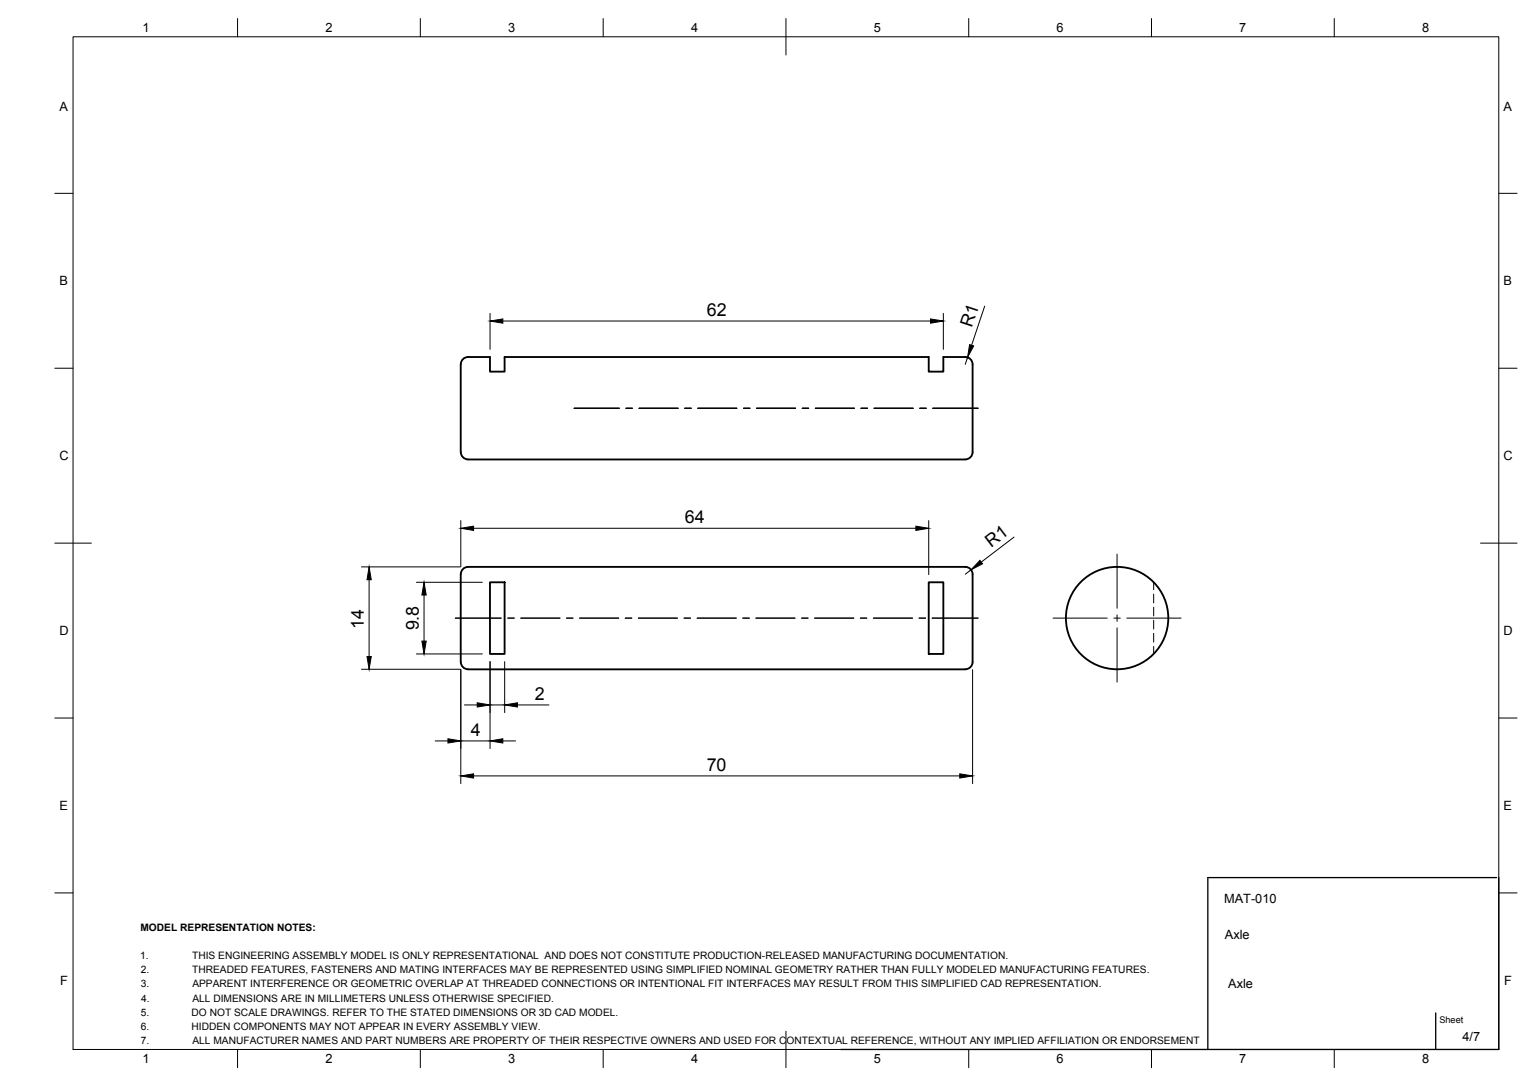
ISO-10303-21;
HEADER;
/* Generated by software containing ST-Developer
 * from STEP Tools, Inc. (www.steptools.com) 
 */

FILE_DESCRIPTION(
/* description */ ('STEP AP214'),
/* implementation_level */ '2;1');

FILE_NAME(
/* name */ 'Axle.step',
/* time_stamp */ '2026-11-14T05:50:49-08:00',
/* author */ (''),
/* organization */ (''),
/* preprocessor_version */ 'ST-DEVELOPER v20.2',
/* originating_system */ 'Autodesk Translation Framework v15.17.0.0',
/* authorisation */ '');

FILE_SCHEMA (('AUTOMOTIVE_DESIGN { 1 0 10303 214 3 1 1 }'));
ENDSEC;

DATA;
#10=MECHANICAL_DESIGN_GEOMETRIC_PRESENTATION_REPRESENTATION('',(#158),#9903);
#134=TOROIDAL_SURFACE('',#2118,6.,1.);
#135=TOROIDAL_SURFACE('',#2123,6.,1.);
#144=SHAPE_REPRESENTATION_RELATIONSHIP('SRR','None',#9939,#151);
#151=ADVANCED_BREP_SHAPE_REPRESENTATION('',(#165),#9897);
#158=STYLED_ITEM('',(#9983),#165);
#165=MANIFOLD_SOLID_BREP('Body1',#2023);
#173=FACE_BOUND('',#379,.T.);
#174=FACE_BOUND('',#380,.T.);
#198=PLANE('',#2133);
#199=PLANE('',#2134);
#200=PLANE('',#2135);
#201=PLANE('',#2136);
#202=PLANE('',#2137);
#203=PLANE('',#2138);
#204=PLANE('',#2139);
#205=PLANE('',#2140);
#256=FACE_OUTER_BOUND('',#376,.T.);
#257=FACE_OUTER_BOUND('',#377,.T.);
#258=FACE_OUTER_BOUND('',#378,.T.);
#259=FACE_OUTER_BOUND('',#381,.T.);
#260=FACE_OUTER_BOUND('',#382,.T.);
#261=FACE_OUTER_BOUND('',#383,.T.);
#262=FACE_OUTER_BOUND('',#384,.T.);
#263=FACE_OUTER_BOUND('',#385,.T.);
#264=FACE_OUTER_BOUND('',#386,.T.);
#265=FACE_OUTER_BOUND('',#387,.T.);
#266=FACE_OUTER_BOUND('',#388,.T.);
#376=EDGE_LOOP('',(#1322,#1323,#1324,#1325,#1326));
#377=EDGE_LOOP('',(#1327,#1328,#1329,#1330,#1331));
#378=EDGE_LOOP('',(#1332,#1333,#1334,#1335,#1336,#1337));
#379=EDGE_LOOP('',(#1338,#1339,#1340,#1341));
#380=EDGE_LOOP('',(#1342,#1343,#1344,#1345));
#381=EDGE_LOOP('',(#1346));
#382=EDGE_LOOP('',(#1347));
#383=EDGE_LOOP('',(#1348,#1349,#1350,#1351));
#384=EDGE_LOOP('',(#1352,#1353));
#385=EDGE_LOOP('',(#1354,#1355));
#386=EDGE_LOOP('',(#1356,#1357,#1358,#1359));
#387=EDGE_LOOP('',(#1360,#1361));
#388=EDGE_LOOP('',(#1362,#1363));
#515=LINE('',#2910,#651);
#516=LINE('',#2913,#652);
#517=LINE('',#2917,#653);
#518=LINE('',#2921,#654);
#519=LINE('',#2925,#655);
#520=LINE('',#2930,#656);
#521=LINE('',#2931,#657);
#522=LINE('',#2935,#658);
#523=LINE('',#2936,#659);
#651=VECTOR('',#2364,7.);
#652=VECTOR('',#2365,1000.);
#653=VECTOR('',#2368,1000.);
#654=VECTOR('',#2371,1000.);
#655=VECTOR('',#2374,1000.);
#656=VECTOR('',#2383,1000.);
#657=VECTOR('',#2384,1000.);
#658=VECTOR('',#2391,1000.);
#659=VECTOR('',#2392,1000.);
#789=CIRCLE('',#2119,6.);
#790=CIRCLE('',#2120,1.);
#791=CIRCLE('',#2121,7.);
#792=CIRCLE('',#2122,7.);
#793=CIRCLE('',#2124,7.);
#794=CIRCLE('',#2125,7.);
#795=CIRCLE('',#2126,1.);
#796=CIRCLE('',#2127,6.);
#797=CIRCLE('',#2129,7.);
#798=CIRCLE('',#2130,7.);
#799=CIRCLE('',#2131,7.);
#800=CIRCLE('',#2132,7.);
#863=VERTEX_POINT('',#2894);
#864=VERTEX_POINT('',#2896);
#865=VERTEX_POINT('',#2898);
#866=VERTEX_POINT('',#2902);
#867=VERTEX_POINT('',#2903);
#868=VERTEX_POINT('',#2906);
#869=VERTEX_POINT('',#2911);
#870=VERTEX_POINT('',#2912);
#871=VERTEX_POINT('',#2914);
#872=VERTEX_POINT('',#2916);
#873=VERTEX_POINT('',#2919);
#874=VERTEX_POINT('',#2920);
#875=VERTEX_POINT('',#2922);
#876=VERTEX_POINT('',#2924);
#1042=EDGE_CURVE('',#863,#863,#789,.T.);
#1043=EDGE_CURVE('',#863,#864,#790,.T.);
#1044=EDGE_CURVE('',#865,#864,#791,.T.);
#1045=EDGE_CURVE('',#864,#865,#792,.T.);
#1046=EDGE_CURVE('',#866,#867,#793,.T.);
#1047=EDGE_CURVE('',#867,#866,#794,.T.);
#1048=EDGE_CURVE('',#867,#868,#795,.T.);
#1049=EDGE_CURVE('',#868,#868,#796,.T.);
#1050=EDGE_CURVE('',#866,#865,#515,.T.);
#1051=EDGE_CURVE('',#869,#870,#516,.T.);
#1052=EDGE_CURVE('',#869,#871,#797,.T.);
#1053=EDGE_CURVE('',#872,#871,#517,.T.);
#1054=EDGE_CURVE('',#870,#872,#798,.T.);
#1055=EDGE_CURVE('',#873,#874,#518,.T.);
#1056=EDGE_CURVE('',#873,#875,#799,.T.);
#1057=EDGE_CURVE('',#876,#875,#519,.T.);
#1058=EDGE_CURVE('',#874,#876,#800,.T.);
#1059=EDGE_CURVE('',#876,#874,#520,.T.);
#1060=EDGE_CURVE('',#875,#873,#521,.T.);
#1061=EDGE_CURVE('',#871,#869,#522,.T.);
#1062=EDGE_CURVE('',#872,#870,#523,.T.);
#1322=ORIENTED_EDGE('',*,*,#1042,.F.);
#1323=ORIENTED_EDGE('',*,*,#1043,.T.);
#1324=ORIENTED_EDGE('',*,*,#1044,.F.);
#1325=ORIENTED_EDGE('',*,*,#1045,.F.);
#1326=ORIENTED_EDGE('',*,*,#1043,.F.);
#1327=ORIENTED_EDGE('',*,*,#1046,.F.);
#1328=ORIENTED_EDGE('',*,*,#1047,.F.);
#1329=ORIENTED_EDGE('',*,*,#1048,.T.);
#1330=ORIENTED_EDGE('',*,*,#1049,.F.);
#1331=ORIENTED_EDGE('',*,*,#1048,.F.);
#1332=ORIENTED_EDGE('',*,*,#1046,.T.);
#1333=ORIENTED_EDGE('',*,*,#1047,.T.);
#1334=ORIENTED_EDGE('',*,*,#1050,.T.);
#1335=ORIENTED_EDGE('',*,*,#1044,.T.);
#1336=ORIENTED_EDGE('',*,*,#1045,.T.);
#1337=ORIENTED_EDGE('',*,*,#1050,.F.);
#1338=ORIENTED_EDGE('',*,*,#1051,.F.);
#1339=ORIENTED_EDGE('',*,*,#1052,.T.);
#1340=ORIENTED_EDGE('',*,*,#1053,.F.);
#1341=ORIENTED_EDGE('',*,*,#1054,.F.);
#1342=ORIENTED_EDGE('',*,*,#1055,.F.);
#1343=ORIENTED_EDGE('',*,*,#1056,.T.);
#1344=ORIENTED_EDGE('',*,*,#1057,.F.);
#1345=ORIENTED_EDGE('',*,*,#1058,.F.);
#1346=ORIENTED_EDGE('',*,*,#1042,.T.);
#1347=ORIENTED_EDGE('',*,*,#1049,.T.);
#1348=ORIENTED_EDGE('',*,*,#1055,.T.);
#1349=ORIENTED_EDGE('',*,*,#1059,.F.);
#1350=ORIENTED_EDGE('',*,*,#1057,.T.);
#1351=ORIENTED_EDGE('',*,*,#1060,.T.);
#1352=ORIENTED_EDGE('',*,*,#1060,.F.);
#1353=ORIENTED_EDGE('',*,*,#1056,.F.);
#1354=ORIENTED_EDGE('',*,*,#1059,.T.);
#1355=ORIENTED_EDGE('',*,*,#1058,.T.);
#1356=ORIENTED_EDGE('',*,*,#1053,.T.);
#1357=ORIENTED_EDGE('',*,*,#1061,.T.);
#1358=ORIENTED_EDGE('',*,*,#1051,.T.);
#1359=ORIENTED_EDGE('',*,*,#1062,.F.);
#1360=ORIENTED_EDGE('',*,*,#1061,.F.);
#1361=ORIENTED_EDGE('',*,*,#1052,.F.);
#1362=ORIENTED_EDGE('',*,*,#1062,.T.);
#1363=ORIENTED_EDGE('',*,*,#1054,.T.);
#1860=CYLINDRICAL_SURFACE('',#2128,7.);
#1908=ADVANCED_FACE('',(#256),#134,.T.);
#1909=ADVANCED_FACE('',(#257),#135,.T.);
#1910=ADVANCED_FACE('',(#258,#173,#174),#1860,.T.);
#1911=ADVANCED_FACE('',(#259),#198,.T.);
#1912=ADVANCED_FACE('',(#260),#199,.F.);
#1913=ADVANCED_FACE('',(#261),#200,.T.);
#1914=ADVANCED_FACE('',(#262),#201,.F.);
#1915=ADVANCED_FACE('',(#263),#202,.T.);
#1916=ADVANCED_FACE('',(#264),#203,.T.);
#1917=ADVANCED_FACE('',(#265),#204,.F.);
#1918=ADVANCED_FACE('',(#266),#205,.T.);
#2023=CLOSED_SHELL('',(#1908,#1909,#1910,#1911,#1912,#1913,#1914,#1915,
#1916,#1917,#1918));
#2117=AXIS2_PLACEMENT_3D('',#2892,#2340,#2341);
#2118=AXIS2_PLACEMENT_3D('',#2893,#2342,#2343);
#2119=AXIS2_PLACEMENT_3D('',#2895,#2344,#2345);
#2120=AXIS2_PLACEMENT_3D('',#2897,#2346,#2347);
#2121=AXIS2_PLACEMENT_3D('',#2899,#2348,#2349);
#2122=AXIS2_PLACEMENT_3D('',#2900,#2350,#2351);
#2123=AXIS2_PLACEMENT_3D('',#2901,#2352,#2353);
#2124=AXIS2_PLACEMENT_3D('',#2904,#2354,#2355);
#2125=AXIS2_PLACEMENT_3D('',#2905,#2356,#2357);
#2126=AXIS2_PLACEMENT_3D('',#2907,#2358,#2359);
#2127=AXIS2_PLACEMENT_3D('',#2908,#2360,#2361);
#2128=AXIS2_PLACEMENT_3D('',#2909,#2362,#2363);
#2129=AXIS2_PLACEMENT_3D('',#2915,#2366,#2367);
#2130=AXIS2_PLACEMENT_3D('',#2918,#2369,#2370);
#2131=AXIS2_PLACEMENT_3D('',#2923,#2372,#2373);
#2132=AXIS2_PLACEMENT_3D('',#2926,#2375,#2376);
#2133=AXIS2_PLACEMENT_3D('',#2927,#2377,#2378);
#2134=AXIS2_PLACEMENT_3D('',#2928,#2379,#2380);
#2135=AXIS2_PLACEMENT_3D('',#2929,#2381,#2382);
#2136=AXIS2_PLACEMENT_3D('',#2932,#2385,#2386);
#2137=AXIS2_PLACEMENT_3D('',#2933,#2387,#2388);
#2138=AXIS2_PLACEMENT_3D('',#2934,#2389,#2390);
#2139=AXIS2_PLACEMENT_3D('',#2937,#2393,#2394);
#2140=AXIS2_PLACEMENT_3D('',#2938,#2395,#2396);
#2340=DIRECTION('axis',(0.,0.,1.));
#2341=DIRECTION('refdir',(1.,0.,0.));
#2342=DIRECTION('center_axis',(0.,0.,1.));
#2343=DIRECTION('ref_axis',(1.,0.,0.));
#2344=DIRECTION('center_axis',(0.,0.,1.));
#2345=DIRECTION('ref_axis',(1.,0.,0.));
#2346=DIRECTION('center_axis',(1.22464679914735E-16,-1.,0.));
#2347=DIRECTION('ref_axis',(-1.,-1.22464679914735E-16,0.));
#2348=DIRECTION('center_axis',(0.,0.,-1.));
#2349=DIRECTION('ref_axis',(1.,0.,0.));
#2350=DIRECTION('center_axis',(0.,0.,-1.));
#2351=DIRECTION('ref_axis',(1.,0.,0.));
#2352=DIRECTION('center_axis',(0.,0.,1.));
#2353=DIRECTION('ref_axis',(1.,0.,0.));
#2354=DIRECTION('center_axis',(0.,0.,1.));
#2355=DIRECTION('ref_axis',(1.,0.,0.));
#2356=DIRECTION('center_axis',(0.,0.,1.));
#2357=DIRECTION('ref_axis',(1.,0.,0.));
#2358=DIRECTION('center_axis',(1.22464679914735E-16,-1.,0.));
#2359=DIRECTION('ref_axis',(-1.,-1.22464679914735E-16,0.));
#2360=DIRECTION('center_axis',(0.,0.,-1.));
#2361=DIRECTION('ref_axis',(1.,0.,0.));
#2362=DIRECTION('center_axis',(0.,0.,-1.));
#2363=DIRECTION('ref_axis',(-1.,0.,0.));
#2364=DIRECTION('',(0.,0.,1.));
#2365=DIRECTION('',(0.,0.,1.));
#2366=DIRECTION('center_axis',(0.,0.,-1.));
#2367=DIRECTION('ref_axis',(-1.,0.,0.));
#2368=DIRECTION('',(0.,0.,-1.));
#2369=DIRECTION('center_axis',(0.,0.,-1.));
#2370=DIRECTION('ref_axis',(-1.,0.,0.));
#2371=DIRECTION('',(0.,0.,-1.));
#2372=DIRECTION('center_axis',(0.,0.,1.));
#2373=DIRECTION('ref_axis',(1.,0.,0.));
#2374=DIRECTION('',(0.,0.,1.));
#2375=DIRECTION('center_axis',(0.,0.,1.));
#2376=DIRECTION('ref_axis',(1.,0.,0.));
#2377=DIRECTION('center_axis',(0.,0.,1.));
#2378=DIRECTION('ref_axis',(1.,0.,0.));
#2379=DIRECTION('center_axis',(0.,0.,1.));
#2380=DIRECTION('ref_axis',(1.,0.,0.));
#2381=DIRECTION('center_axis',(0.,1.,0.));
#2382=DIRECTION('ref_axis',(0.,0.,1.));
#2383=DIRECTION('',(1.,0.,0.));
#2384=DIRECTION('',(1.,0.,0.));
#2385=DIRECTION('center_axis',(0.,0.,1.));
#2386=DIRECTION('ref_axis',(1.,0.,0.));
#2387=DIRECTION('center_axis',(0.,0.,1.));
#2388=DIRECTION('ref_axis',(1.,0.,0.));
#2389=DIRECTION('center_axis',(0.,1.,0.));
#2390=DIRECTION('ref_axis',(0.,0.,1.));
#2391=DIRECTION('',(-1.,0.,0.));
#2392=DIRECTION('',(-1.,0.,0.));
#2393=DIRECTION('center_axis',(0.,0.,-1.));
#2394=DIRECTION('ref_axis',(-1.,0.,0.));
#2395=DIRECTION('center_axis',(0.,0.,-1.));
#2396=DIRECTION('ref_axis',(-1.,0.,0.));
#2892=CARTESIAN_POINT('',(0.,0.,0.));
#2893=CARTESIAN_POINT('Origin',(0.,0.,69.));
#2894=CARTESIAN_POINT('',(-6.,-7.34788079488412E-16,70.));
#2895=CARTESIAN_POINT('Origin',(0.,0.,70.));
#2896=CARTESIAN_POINT('',(-7.,-8.57252759403147E-16,69.));
#2897=CARTESIAN_POINT('Origin',(-6.,-7.34788079488412E-16,69.));
#2898=CARTESIAN_POINT('',(7.,8.57252759403147E-16,69.));
#2899=CARTESIAN_POINT('Origin',(0.,0.,69.));
#2900=CARTESIAN_POINT('Origin',(0.,0.,69.));
#2901=CARTESIAN_POINT('Origin',(0.,0.,1.));
#2902=CARTESIAN_POINT('',(7.,8.57252759403147E-16,1.));
#2903=CARTESIAN_POINT('',(-7.,-8.57252759403147E-16,1.));
#2904=CARTESIAN_POINT('Origin',(0.,0.,1.));
#2905=CARTESIAN_POINT('Origin',(0.,0.,1.));
#2906=CARTESIAN_POINT('',(-6.,-7.34788079488412E-16,0.));
#2907=CARTESIAN_POINT('Origin',(-6.,-7.34788079488412E-16,1.));
#2908=CARTESIAN_POINT('Origin',(0.,0.,0.));
#2909=CARTESIAN_POINT('Origin',(0.,0.,70.));
#2910=CARTESIAN_POINT('',(7.,-8.57252759403147E-16,70.));
#2911=CARTESIAN_POINT('',(-4.89897948556636,5.,4.));
#2912=CARTESIAN_POINT('',(-4.89897948556636,5.,6.00000000000001));
#2913=CARTESIAN_POINT('',(-4.89897948556636,5.,70.));
#2914=CARTESIAN_POINT('',(4.89897948556636,5.,4.));
#2915=CARTESIAN_POINT('Origin',(0.,0.,4.));
#2916=CARTESIAN_POINT('',(4.89897948556636,5.,6.00000000000001));
#2917=CARTESIAN_POINT('',(4.89897948556636,5.,70.));
#2918=CARTESIAN_POINT('Origin',(0.,0.,6.00000000000001));
#2919=CARTESIAN_POINT('',(4.89897948556636,5.,66.));
#2920=CARTESIAN_POINT('',(4.89897948556636,5.,64.));
#2921=CARTESIAN_POINT('',(4.89897948556636,5.,70.));
#2922=CARTESIAN_POINT('',(-4.89897948556636,5.,66.));
#2923=CARTESIAN_POINT('Origin',(0.,0.,66.));
#2924=CARTESIAN_POINT('',(-4.89897948556636,5.,64.));
#2925=CARTESIAN_POINT('',(-4.89897948556636,5.,70.));
#2926=CARTESIAN_POINT('Origin',(0.,0.,64.));
#2927=CARTESIAN_POINT('Origin',(0.,0.,70.));
#2928=CARTESIAN_POINT('Origin',(0.,0.,0.));
#2929=CARTESIAN_POINT('Origin',(2.44929359829471E-16,5.,66.));
#2930=CARTESIAN_POINT('',(2.44929359829471E-16,5.,64.));
#2931=CARTESIAN_POINT('',(-6.13964394045187,5.,66.));
#2932=CARTESIAN_POINT('Origin',(0.,0.,66.));
#2933=CARTESIAN_POINT('Origin',(0.,0.,64.));
#2934=CARTESIAN_POINT('Origin',(-2.44929359829471E-16,5.,4.));
#2935=CARTESIAN_POINT('',(5.87651634300394,5.,4.));
#2936=CARTESIAN_POINT('',(-2.44929359829471E-16,5.,6.));
#2937=CARTESIAN_POINT('Origin',(0.,0.,4.));
#2938=CARTESIAN_POINT('Origin',(0.,0.,6.));
#9888=UNCERTAINTY_MEASURE_WITH_UNIT(LENGTH_MEASURE(0.01),#9904,
'DISTANCE_ACCURACY_VALUE',
'Maximum model space distance between geometric entities at asserted c
onnectivities');
#9894=UNCERTAINTY_MEASURE_WITH_UNIT(LENGTH_MEASURE(0.01),#9904,
'DISTANCE_ACCURACY_VALUE',
'Maximum model space distance between geometric entities at asserted c
onnectivities');
#9897=(
GEOMETRIC_REPRESENTATION_CONTEXT(3)
GLOBAL_UNCERTAINTY_ASSIGNED_CONTEXT((#9888))
GLOBAL_UNIT_ASSIGNED_CONTEXT((#9904,#9906,#9907))
REPRESENTATION_CONTEXT('','3D')
);
#9903=(
GEOMETRIC_REPRESENTATION_CONTEXT(3)
GLOBAL_UNCERTAINTY_ASSIGNED_CONTEXT((#9894))
GLOBAL_UNIT_ASSIGNED_CONTEXT((#9904,#9906,#9907))
REPRESENTATION_CONTEXT('','3D')
);
#9904=(
LENGTH_UNIT()
NAMED_UNIT(*)
SI_UNIT(.MILLI.,.METRE.)
);
#9906=(
NAMED_UNIT(*)
PLANE_ANGLE_UNIT()
SI_UNIT($,.RADIAN.)
);
#9907=(
NAMED_UNIT(*)
SI_UNIT($,.STERADIAN.)
SOLID_ANGLE_UNIT()
);
#9910=SHAPE_DEFINITION_REPRESENTATION(#9918,#9939);
#9918=PRODUCT_DEFINITION_SHAPE('',$,#9948);
#9939=SHAPE_REPRESENTATION('',(#2117),#9897);
#9945=PRODUCT_DEFINITION_CONTEXT('part definition',#9971,'design');
#9948=PRODUCT_DEFINITION('Axle','Axle',#9956,#9945);
#9956=PRODUCT_DEFINITION_FORMATION('',$,#9975);
#9971=APPLICATION_CONTEXT(
'Core Data for Automotive Mechanical Design Process');
#9972=PRODUCT_CONTEXT('part definition',#9971,'mechanical');
#9975=PRODUCT('Axle','Axle',$,(#9972));
#9983=PRESENTATION_STYLE_ASSIGNMENT((#9988));
#9988=SURFACE_STYLE_USAGE(.BOTH.,#9993);
#9993=SURFACE_SIDE_STYLE('',(#9998));
#9998=SURFACE_STYLE_FILL_AREA(#10003);
#10003=FILL_AREA_STYLE('Opaque(61,176,222)',(#10008));
#10008=FILL_AREA_STYLE_COLOUR('Opaque(61,176,222)',#10013);
#10013=COLOUR_RGB('Opaque(61,176,222)',0.23921568627451,0.690196078431373,
0.870588235294118);
ENDSEC;
END-ISO-10303-21;
